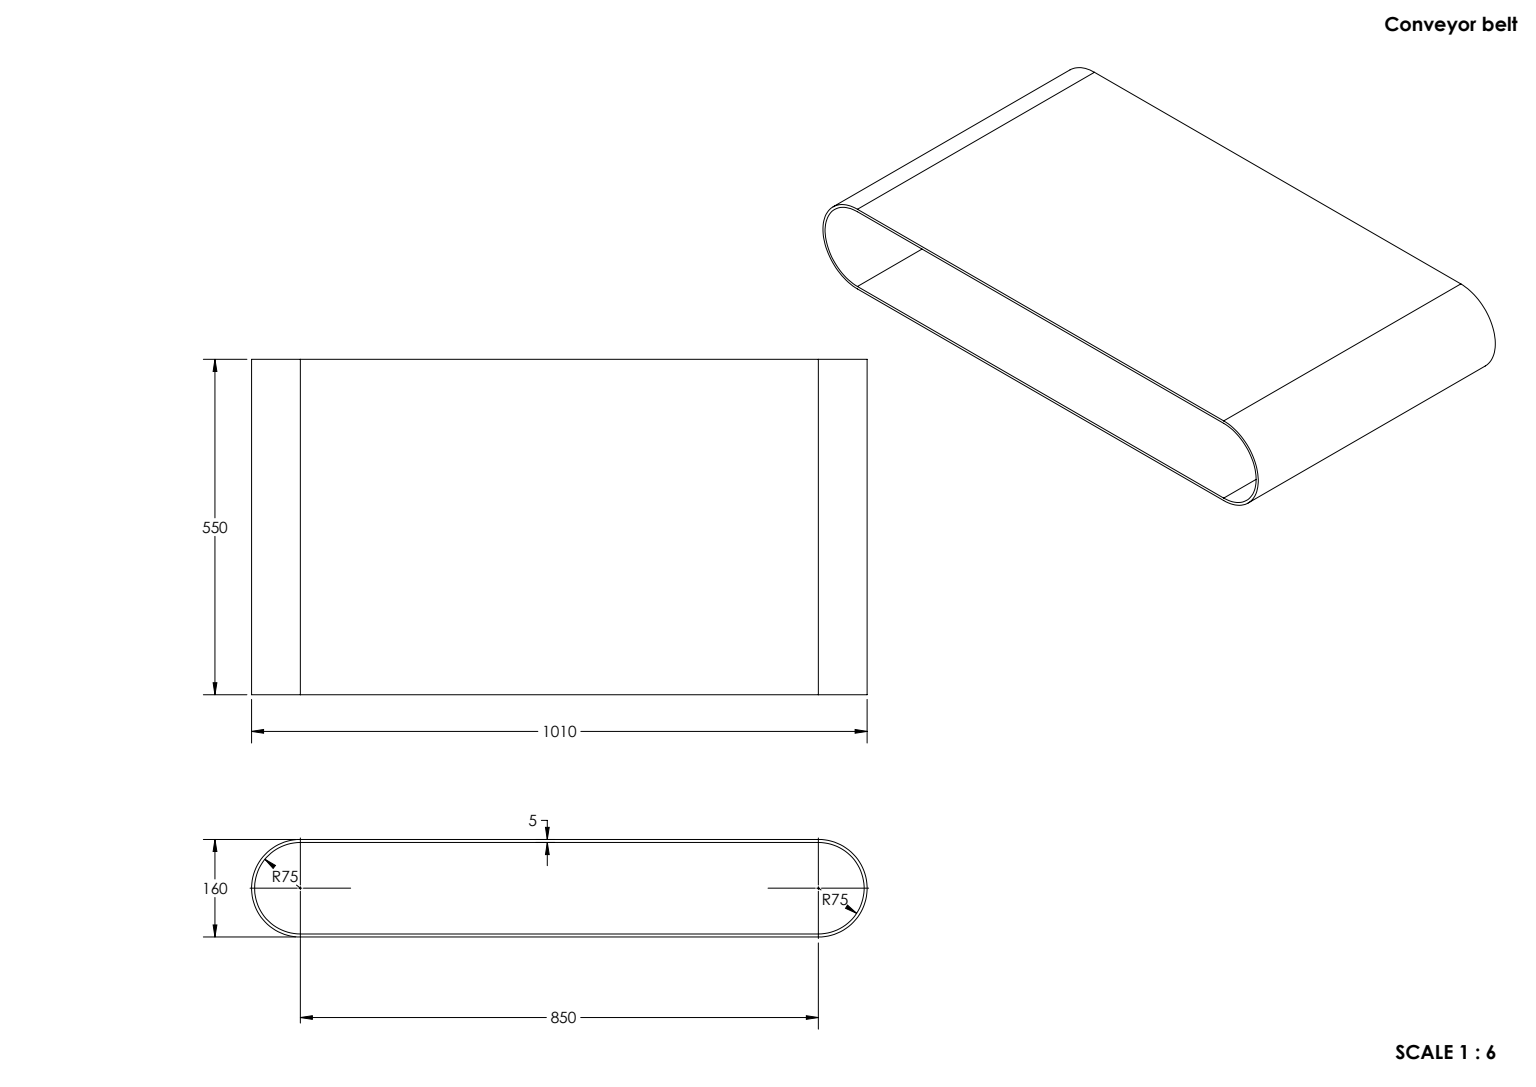
ISO-10303-21;
HEADER;
FILE_DESCRIPTION (('STEP AP214'),
    '1' );
FILE_NAME ('Conveyor belt.step',
    '2026-10-24T15:53:57',
    ( '' ),
    ( '' ),
    'SwSTEP 2.0',
    'SolidWorks 2025',
    '' );
FILE_SCHEMA (( 'AUTOMOTIVE_DESIGN' ));
ENDSEC;

DATA;
#9=LINE ( 'NONE', #1201, #6141 ) ;
#21=VERTEX_POINT ( 'NONE', #2818 ) ;
#37=PRODUCT_CONTEXT ( 'NONE', #2802, 'mechanical' ) ;
#53=CARTESIAN_POINT ( 'NONE',  ( 275.0000000000000000, -425.0000000000000000, 80.00000000000000000 ) ) ;
#85=ORIENTED_EDGE ( 'NONE', *, *, #6307, .F. ) ;
#150=( NAMED_UNIT ( * ) PLANE_ANGLE_UNIT ( ) SI_UNIT ( $, .RADIAN. ) );
#157=CYLINDRICAL_SURFACE ( 'NONE', #5418, 80.00000000000000000 ) ;
#189=AXIS2_PLACEMENT_3D ( 'NONE', #4605, #682, #3336 ) ;
#195=( NAMED_UNIT ( * ) SI_UNIT ( $, .STERADIAN. ) SOLID_ANGLE_UNIT ( ) );
#211=CARTESIAN_POINT ( 'NONE',  ( -275.0000000000000000, -425.0000000000000000, 75.00000000000000000 ) ) ;
#230=ADVANCED_BREP_SHAPE_REPRESENTATION ( '', ( #2980, #7563 ), #1574 ) ;
#257=ORIENTED_EDGE ( 'NONE', *, *, #5557, .F. ) ;
#285=( GEOMETRIC_REPRESENTATION_CONTEXT ( 3 ) GLOBAL_UNCERTAINTY_ASSIGNED_CONTEXT ( ( #4742 ) ) GLOBAL_UNIT_ASSIGNED_CONTEXT ( ( #5304, #150, #6149 ) ) REPRESENTATION_CONTEXT ( 'NONE', 'WORKASPACE' ) );
#287=AXIS2_PLACEMENT_3D ( 'NONE', #7730, #8435, #429 ) ;
#329=ORIENTED_EDGE ( 'NONE', *, *, #2161, .T. ) ;
#356=VECTOR ( 'NONE', #2554, 1000.000000000000000 ) ;
#429=DIRECTION ( 'NONE',  ( 0.000000000000000000, 0.000000000000000000, -1.000000000000000000 ) ) ;
#443=ORIENTED_EDGE ( 'NONE', *, *, #4512, .F. ) ;
#457=CIRCLE ( 'NONE', #6440, 80.00000000000001421 ) ;
#520=DIRECTION ( 'NONE',  ( 0.000000000000000000, 0.000000000000000000, -1.000000000000000000 ) ) ;
#571=EDGE_CURVE ( 'NONE', #3965, #8336, #5577, .T. ) ;
#579=VERTEX_POINT ( 'NONE', #822 ) ;
#614=CARTESIAN_POINT ( 'NONE',  ( 275.0000000000000000, 425.0000000000000000, 1.561424668912875158E-13 ) ) ;
#620=SHAPE_DEFINITION_REPRESENTATION ( #629, #5209 ) ;
#629=PRODUCT_DEFINITION_SHAPE ( 'NONE', 'NONE',  #2753 ) ;
#644=CARTESIAN_POINT ( 'NONE',  ( -275.0000000000000000, 425.0000000000000000, 75.00000000000015632 ) ) ;
#682=DIRECTION ( 'NONE',  ( -1.000000000000000000, -0.000000000000000000, -0.000000000000000000 ) ) ;
#684=ADVANCED_FACE ( 'NONE', ( #8308 ), #1670, .T. ) ;
#700=DIRECTION ( 'NONE',  ( -1.000000000000000000, -0.000000000000000000, -0.000000000000000000 ) ) ;
#793=CIRCLE ( 'NONE', #2448, 80.00000000000001421 ) ;
#804=ORIENTED_EDGE ( 'NONE', *, *, #5681, .F. ) ;
#822=CARTESIAN_POINT ( 'NONE',  ( 275.0000000000000000, 425.0000000000000000, -74.99999999999984368 ) ) ;
#828=VERTEX_POINT ( 'NONE', #1919 ) ;
#852=DIRECTION ( 'NONE',  ( 1.000000000000000000, 0.000000000000000000, 0.000000000000000000 ) ) ;
#877=DIRECTION ( 'NONE',  ( -1.000000000000000000, -0.000000000000000000, -0.000000000000000000 ) ) ;
#897=AXIS2_PLACEMENT_3D ( 'NONE', #2889, #852, #2808 ) ;
#937=FACE_OUTER_BOUND ( 'NONE', #8273, .T. ) ;
#966=VECTOR ( 'NONE', #3191, 1000.000000000000000 ) ;
#975=CARTESIAN_POINT ( 'NONE',  ( 275.0000000000000000, -425.0000000000000000, 80.00000000000000000 ) ) ;
#985=EDGE_CURVE ( 'NONE', #2467, #3965, #3106, .T. ) ;
#1037=ORIENTED_EDGE ( 'NONE', *, *, #5557, .T. ) ;
#1062=EDGE_CURVE ( 'NONE', #828, #3789, #4177, .T. ) ;
#1077=ADVANCED_FACE ( 'NONE', ( #2263 ), #4920, .T. ) ;
#1090=PLANE ( 'NONE',  #1105 ) ;
#1105=AXIS2_PLACEMENT_3D ( 'NONE', #1685, #4478, #520 ) ;
#1121=DIRECTION ( 'NONE',  ( 0.000000000000000000, -1.000000000000000000, -1.795949010423047620E-16 ) ) ;
#1122=EDGE_LOOP ( 'NONE', ( #2153, #1445, #329, #3321 ) ) ;
#1124=EDGE_CURVE ( 'NONE', #8386, #828, #1181, .T. ) ;
#1168=FACE_OUTER_BOUND ( 'NONE', #1171, .T. ) ;
#1171=EDGE_LOOP ( 'NONE', ( #804, #4109, #3770, #257 ) ) ;
#1181=CIRCLE ( 'NONE', #6081, 80.00000000000001421 ) ;
#1193=VECTOR ( 'NONE', #3510, 1000.000000000000000 ) ;
#1201=CARTESIAN_POINT ( 'NONE',  ( 275.0000000000000000, 425.0000000000000000, 80.00000000000015632 ) ) ;
#1283=PLANE ( 'NONE',  #3713 ) ;
#1286=CARTESIAN_POINT ( 'NONE',  ( -275.0000000000000000, -425.0000000000000000, -75.00000000000000000 ) ) ;
#1328=EDGE_CURVE ( 'NONE', #828, #6748, #1386, .T. ) ;
#1339=UNCERTAINTY_MEASURE_WITH_UNIT (LENGTH_MEASURE( 1.000000000000000082E-05 ), #2325, 'distance_accuracy_value', 'NONE');
#1369=ORIENTED_EDGE ( 'NONE', *, *, #4136, .F. ) ;
#1386=LINE ( 'NONE', #4044, #8427 ) ;
#1426=LINE ( 'NONE', #2771, #1193 ) ;
#1436=ORIENTED_EDGE ( 'NONE', *, *, #5113, .F. ) ;
#1445=ORIENTED_EDGE ( 'NONE', *, *, #8307, .F. ) ;
#1526=EDGE_CURVE ( 'NONE', #6748, #2467, #4507, .T. ) ;
#1574=( GEOMETRIC_REPRESENTATION_CONTEXT ( 3 ) GLOBAL_UNCERTAINTY_ASSIGNED_CONTEXT ( ( #1339 ) ) GLOBAL_UNIT_ASSIGNED_CONTEXT ( ( #2325, #6916, #195 ) ) REPRESENTATION_CONTEXT ( 'NONE', 'WORKASPACE' ) );
#1576=AXIS2_PLACEMENT_3D ( 'NONE', #7579, #7742, #2468 ) ;
#1581=ORIENTED_EDGE ( 'NONE', *, *, #5507, .T. ) ;
#1595=DIRECTION ( 'NONE',  ( 0.000000000000000000, -1.000000000000000000, -1.795949010423047620E-16 ) ) ;
#1600=ORIENTED_EDGE ( 'NONE', *, *, #1062, .F. ) ;
#1609=VECTOR ( 'NONE', #4423, 1000.000000000000000 ) ;
#1670=CYLINDRICAL_SURFACE ( 'NONE', #5189, 80.00000000000000000 ) ;
#1676=CARTESIAN_POINT ( 'NONE',  ( 275.0000000000000000, 425.0000000000000000, 75.00000000000015632 ) ) ;
#1685=CARTESIAN_POINT ( 'NONE',  ( -275.0000000000000000, -425.0000000000000000, 0.000000000000000000 ) ) ;
#1755=ADVANCED_FACE ( 'NONE', ( #2731 ), #1283, .F. ) ;
#1858=VECTOR ( 'NONE', #877, 1000.000000000000000 ) ;
#1868=EDGE_LOOP ( 'NONE', ( #443, #5994, #2835, #8154 ) ) ;
#1919=CARTESIAN_POINT ( 'NONE',  ( 275.0000000000000000, -425.0000000000000000, -80.00000000000000000 ) ) ;
#1994=CARTESIAN_POINT ( 'NONE',  ( -275.0000000000000000, -425.0000000000000000, 0.000000000000000000 ) ) ;
#2043=ORIENTED_EDGE ( 'NONE', *, *, #5848, .T. ) ;
#2051=EDGE_CURVE ( 'NONE', #2597, #579, #5794, .T. ) ;
#2153=ORIENTED_EDGE ( 'NONE', *, *, #2377, .F. ) ;
#2161=EDGE_CURVE ( 'NONE', #4536, #8239, #6044, .T. ) ;
#2203=ORIENTED_EDGE ( 'NONE', *, *, #3116, .T. ) ;
#2206=SHAPE_REPRESENTATION_RELATIONSHIP ( 'NONE' , 'NONE' ,  #5209, #230 ) ;
#2226=EDGE_CURVE ( 'NONE', #8239, #3300, #5651, .T. ) ;
#2227=CARTESIAN_POINT ( 'NONE',  ( 275.0000000000000000, 425.0000000000000000, 75.00000000000015632 ) ) ;
#2229=STYLED_ITEM('',(#8670),#2980);
#2257=EDGE_LOOP ( 'NONE', ( #2795, #7341, #6442, #2605 ) ) ;
#2263=FACE_OUTER_BOUND ( 'NONE', #1122, .T. ) ;
#2296=DIRECTION ( 'NONE',  ( 0.000000000000000000, 0.000000000000000000, 1.000000000000000000 ) ) ;
#2325=( LENGTH_UNIT ( ) NAMED_UNIT ( * ) SI_UNIT ( .MILLI., .METRE. ) );
#2358=FACE_OUTER_BOUND ( 'NONE', #2257, .T. ) ;
#2359=VECTOR ( 'NONE', #8298, 1000.000000000000000 ) ;
#2377=EDGE_CURVE ( 'NONE', #5689, #3300, #4968, .T. ) ;
#2388=ORIENTED_EDGE ( 'NONE', *, *, #985, .T. ) ;
#2448=AXIS2_PLACEMENT_3D ( 'NONE', #1994, #4561, #2518 ) ;
#2467=VERTEX_POINT ( 'NONE', #8202 ) ;
#2468=DIRECTION ( 'NONE',  ( 0.000000000000000000, 1.000000000000000000, 1.795949010423047374E-16 ) ) ;
#2474=EDGE_CURVE ( 'NONE', #6426, #8386, #6945, .T. ) ;
#2478=DIRECTION ( 'NONE',  ( 0.000000000000000000, 0.000000000000000000, -1.000000000000000000 ) ) ;
#2518=DIRECTION ( 'NONE',  ( 0.000000000000000000, 1.000000000000000000, 0.000000000000000000 ) ) ;
#2519=ADVANCED_FACE ( 'NONE', ( #2804 ), #3500, .T. ) ;
#2554=DIRECTION ( 'NONE',  ( 0.000000000000000000, 1.000000000000000000, 1.795949010423047374E-16 ) ) ;
#2589=ORIENTED_EDGE ( 'NONE', *, *, #2474, .F. ) ;
#2597=VERTEX_POINT ( 'NONE', #3720 ) ;
#2605=ORIENTED_EDGE ( 'NONE', *, *, #4352, .T. ) ;
#2612=DIRECTION ( 'NONE',  ( 1.000000000000000000, 0.000000000000000000, 0.000000000000000000 ) ) ;
#2625=ORIENTED_EDGE ( 'NONE', *, *, #4808, .F. ) ;
#2660=LINE ( 'NONE', #7836, #7682 ) ;
#2661=ORIENTED_EDGE ( 'NONE', *, *, #3116, .F. ) ;
#2690=CYLINDRICAL_SURFACE ( 'NONE', #189, 75.00000000000000000 ) ;
#2708=LINE ( 'NONE', #7274, #6315 ) ;
#2719=CARTESIAN_POINT ( 'NONE',  ( 275.0000000000000000, -425.0000000000000000, 75.00000000000000000 ) ) ;
#2720=ORIENTED_EDGE ( 'NONE', *, *, #4512, .T. ) ;
#2731=FACE_OUTER_BOUND ( 'NONE', #8566, .T. ) ;
#2753=PRODUCT_DEFINITION ( 'UNKNOWN', '', #8136, #5248 ) ;
#2771=CARTESIAN_POINT ( 'NONE',  ( -275.0000000000000000, -425.0000000000000000, -80.00000000000000000 ) ) ;
#2775=ORIENTED_EDGE ( 'NONE', *, *, #5681, .T. ) ;
#2795=ORIENTED_EDGE ( 'NONE', *, *, #5848, .F. ) ;
#2802=APPLICATION_CONTEXT ( 'automotive_design' ) ;
#2804=FACE_OUTER_BOUND ( 'NONE', #6816, .T. ) ;
#2807=ORIENTED_EDGE ( 'NONE', *, *, #2161, .F. ) ;
#2808=DIRECTION ( 'NONE',  ( 0.000000000000000000, 0.000000000000000000, -1.000000000000000000 ) ) ;
#2818=CARTESIAN_POINT ( 'NONE',  ( -275.0000000000000000, 425.0000000000000000, -74.99999999999984368 ) ) ;
#2835=ORIENTED_EDGE ( 'NONE', *, *, #4808, .T. ) ;
#2853=DIRECTION ( 'NONE',  ( 0.000000000000000000, 1.000000000000000000, 0.000000000000000000 ) ) ;
#2889=CARTESIAN_POINT ( 'NONE',  ( 275.0000000000000000, -425.0000000000000000, 0.000000000000000000 ) ) ;
#2897=ORIENTED_EDGE ( 'NONE', *, *, #571, .T. ) ;
#2949=LINE ( 'NONE', #1676, #4319 ) ;
#2978=VERTEX_POINT ( 'NONE', #3338 ) ;
#2980=MANIFOLD_SOLID_BREP ( 'Extrude-Thin1', #6001 ) ;
#2982=CARTESIAN_POINT ( 'NONE',  ( 275.0000000000000000, -425.0000000000000000, 0.000000000000000000 ) ) ;
#2989=EDGE_LOOP ( 'NONE', ( #8204, #85, #2807, #2625 ) ) ;
#3100=CYLINDRICAL_SURFACE ( 'NONE', #4489, 75.00000000000000000 ) ;
#3106=CIRCLE ( 'NONE', #7421, 80.00000000000001421 ) ;
#3116=EDGE_CURVE ( 'NONE', #8386, #8336, #2660, .T. ) ;
#3175=ORIENTED_EDGE ( 'NONE', *, *, #2051, .T. ) ;
#3191=DIRECTION ( 'NONE',  ( -0.000000000000000000, -1.000000000000000000, -1.795949010423047374E-16 ) ) ;
#3234=VECTOR ( 'NONE', #1595, 1000.000000000000000 ) ;
#3239=APPLICATION_CONTEXT ( 'automotive_design' ) ;
#3293=CIRCLE ( 'NONE', #8170, 75.00000000000000000 ) ;
#3299=CARTESIAN_POINT ( 'NONE',  ( 275.0000000000000000, -425.0000000000000000, 75.00000000000000000 ) ) ;
#3300=VERTEX_POINT ( 'NONE', #211 ) ;
#3321=ORIENTED_EDGE ( 'NONE', *, *, #2226, .T. ) ;
#3335=LINE ( 'NONE', #1286, #356 ) ;
#3336=DIRECTION ( 'NONE',  ( 0.000000000000000000, 0.000000000000000000, 1.000000000000000000 ) ) ;
#3338=CARTESIAN_POINT ( 'NONE',  ( -275.0000000000000000, -425.0000000000000000, -75.00000000000000000 ) ) ;
#3367=ORIENTED_EDGE ( 'NONE', *, *, #5113, .T. ) ;
#3411=DIRECTION ( 'NONE',  ( 1.000000000000000000, 0.000000000000000000, 0.000000000000000000 ) ) ;
#3419=PLANE ( 'NONE',  #897 ) ;
#3477=CARTESIAN_POINT ( 'NONE',  ( 275.0000000000000000, 425.0000000000000000, 1.561424668912875158E-13 ) ) ;
#3491=ORIENTED_EDGE ( 'NONE', *, *, #4136, .T. ) ;
#3500=PLANE ( 'NONE',  #6268 ) ;
#3510=DIRECTION ( 'NONE',  ( 0.000000000000000000, 1.000000000000000000, 1.795949010423047620E-16 ) ) ;
#3512=DIRECTION ( 'NONE',  ( 1.000000000000000000, 0.000000000000000000, 0.000000000000000000 ) ) ;
#3514=ORIENTED_EDGE ( 'NONE', *, *, #4352, .F. ) ;
#3569=DIRECTION ( 'NONE',  ( -1.000000000000000000, -0.000000000000000000, -0.000000000000000000 ) ) ;
#3707=DIRECTION ( 'NONE',  ( 1.000000000000000000, 0.000000000000000000, 0.000000000000000000 ) ) ;
#3713=AXIS2_PLACEMENT_3D ( 'NONE', #53, #7557, #5430 ) ;
#3720=CARTESIAN_POINT ( 'NONE',  ( 275.0000000000000000, -425.0000000000000000, -75.00000000000000000 ) ) ;
#3732=CARTESIAN_POINT ( 'NONE',  ( 275.0000000000000000, -425.0000000000000000, 0.000000000000000000 ) ) ;
#3739=LINE ( 'NONE', #6973, #6896 ) ;
#3770=ORIENTED_EDGE ( 'NONE', *, *, #985, .F. ) ;
#3789=VERTEX_POINT ( 'NONE', #4785 ) ;
#3847=CARTESIAN_POINT ( 'NONE',  ( -275.0000000000000000, 425.0000000000000000, 80.00000000000015632 ) ) ;
#3863=CARTESIAN_POINT ( 'NONE',  ( 275.0000000000000000, 425.0000000000000000, -79.99999999999984368 ) ) ;
#3900=FACE_OUTER_BOUND ( 'NONE', #6229, .T. ) ;
#3906=ORIENTED_EDGE ( 'NONE', *, *, #5444, .T. ) ;
#3926=DIRECTION ( 'NONE',  ( -0.000000000000000000, -1.000000000000000000, -1.795949010423047374E-16 ) ) ;
#3930=CIRCLE ( 'NONE', #6183, 75.00000000000000000 ) ;
#3965=VERTEX_POINT ( 'NONE', #3847 ) ;
#4042=MECHANICAL_DESIGN_GEOMETRIC_PRESENTATION_REPRESENTATION('',(#2229),#285);
#4044=CARTESIAN_POINT ( 'NONE',  ( 275.0000000000000000, -425.0000000000000000, -80.00000000000000000 ) ) ;
#4049=ORIENTED_EDGE ( 'NONE', *, *, #1526, .F. ) ;
#4051=EDGE_LOOP ( 'NONE', ( #2043, #1581, #2720, #5798 ) ) ;
#4106=ADVANCED_FACE ( 'NONE', ( #937, #5559 ), #3419, .T. ) ;
#4109=ORIENTED_EDGE ( 'NONE', *, *, #571, .F. ) ;
#4136=EDGE_CURVE ( 'NONE', #6748, #6426, #457, .T. ) ;
#4170=DIRECTION ( 'NONE',  ( -1.000000000000000000, -0.000000000000000000, -0.000000000000000000 ) ) ;
#4177=LINE ( 'NONE', #6848, #1858 ) ;
#4198=ADVANCED_FACE ( 'NONE', ( #2358 ), #3100, .F. ) ;
#4203=CARTESIAN_POINT ( 'NONE',  ( 0.000000000000000000, 0.000000000000000000, 0.000000000000000000 ) ) ;
#4307=ORIENTED_EDGE ( 'NONE', *, *, #1526, .T. ) ;
#4319=VECTOR ( 'NONE', #4170, 1000.000000000000000 ) ;
#4352=EDGE_CURVE ( 'NONE', #2597, #2978, #2708, .T. ) ;
#4407=DIRECTION ( 'NONE',  ( -1.000000000000000000, -0.000000000000000000, -0.000000000000000000 ) ) ;
#4423=DIRECTION ( 'NONE',  ( -1.000000000000000000, -0.000000000000000000, -0.000000000000000000 ) ) ;
#4428=CARTESIAN_POINT ( 'NONE',  ( 275.0000000000000000, -425.0000000000000000, -80.00000000000000000 ) ) ;
#4445=ORIENTED_EDGE ( 'NONE', *, *, #1328, .F. ) ;
#4478=DIRECTION ( 'NONE',  ( 1.000000000000000000, 0.000000000000000000, 0.000000000000000000 ) ) ;
#4489=AXIS2_PLACEMENT_3D ( 'NONE', #2982, #6385, #5018 ) ;
#4495=CARTESIAN_POINT ( 'NONE',  ( 275.0000000000000000, -425.0000000000000000, -75.00000000000000000 ) ) ;
#4507=LINE ( 'NONE', #7010, #1609 ) ;
#4512=EDGE_CURVE ( 'NONE', #21, #5689, #5049, .T. ) ;
#4534=CARTESIAN_POINT ( 'NONE',  ( 275.0000000000000000, -425.0000000000000000, 0.000000000000000000 ) ) ;
#4536=VERTEX_POINT ( 'NONE', #2227 ) ;
#4561=DIRECTION ( 'NONE',  ( 1.000000000000000000, 0.000000000000000000, 0.000000000000000000 ) ) ;
#4605=CARTESIAN_POINT ( 'NONE',  ( 275.0000000000000000, 425.0000000000000000, 1.561424668912875158E-13 ) ) ;
#4662=ORIENTED_EDGE ( 'NONE', *, *, #2474, .T. ) ;
#4742=UNCERTAINTY_MEASURE_WITH_UNIT (LENGTH_MEASURE( 1.000000000000000082E-05 ), #5304, 'distance_accuracy_value', 'NONE');
#4785=CARTESIAN_POINT ( 'NONE',  ( -275.0000000000000000, -425.0000000000000000, -80.00000000000000000 ) ) ;
#4787=AXIS2_PLACEMENT_3D ( 'NONE', #6634, #3411, #6724 ) ;
#4808=EDGE_CURVE ( 'NONE', #579, #4536, #3293, .T. ) ;
#4828=CARTESIAN_POINT ( 'NONE',  ( 275.0000000000000000, -425.0000000000000000, 80.00000000000000000 ) ) ;
#4889=DIRECTION ( 'NONE',  ( 0.000000000000000000, -1.000000000000000000, -1.795949010423047620E-16 ) ) ;
#4920=PLANE ( 'NONE',  #1576 ) ;
#4968=LINE ( 'NONE', #7629, #966 ) ;
#4998=CARTESIAN_POINT ( 'NONE',  ( -275.0000000000000000, 425.0000000000000000, 1.561424668912875158E-13 ) ) ;
#5003=ORIENTED_EDGE ( 'NONE', *, *, #1062, .T. ) ;
#5007=VECTOR ( 'NONE', #4407, 1000.000000000000000 ) ;
#5018=DIRECTION ( 'NONE',  ( 0.000000000000000000, 0.000000000000000000, 1.000000000000000000 ) ) ;
#5049=CIRCLE ( 'NONE', #4787, 75.00000000000000000 ) ;
#5070=ORIENTED_EDGE ( 'NONE', *, *, #5507, .F. ) ;
#5113=EDGE_CURVE ( 'NONE', #6426, #3965, #9, .T. ) ;
#5189=AXIS2_PLACEMENT_3D ( 'NONE', #3732, #5718, #6396 ) ;
#5209=SHAPE_REPRESENTATION ( 'Conveyor belt', ( #7563 ), #1574 ) ;
#5248=PRODUCT_DEFINITION_CONTEXT ( 'detailed design', #3239, 'design' ) ;
#5272=EDGE_LOOP ( 'NONE', ( #2775, #1600, #7986, #2203 ) ) ;
#5294=ADVANCED_FACE ( 'NONE', ( #1168, #7791 ), #1090, .F. ) ;
#5304=( LENGTH_UNIT ( ) NAMED_UNIT ( * ) SI_UNIT ( .MILLI., .METRE. ) );
#5418=AXIS2_PLACEMENT_3D ( 'NONE', #3477, #3569, #2296 ) ;
#5426=DIRECTION ( 'NONE',  ( 1.000000000000000000, 0.000000000000000000, 0.000000000000000000 ) ) ;
#5430=DIRECTION ( 'NONE',  ( 0.000000000000000000, 1.000000000000000000, 1.795949010423047620E-16 ) ) ;
#5432=EDGE_LOOP ( 'NONE', ( #2388, #1436, #1369, #4307 ) ) ;
#5444=EDGE_CURVE ( 'NONE', #579, #21, #3739, .T. ) ;
#5507=EDGE_CURVE ( 'NONE', #2978, #21, #3335, .T. ) ;
#5557=EDGE_CURVE ( 'NONE', #3789, #2467, #1426, .T. ) ;
#5559=FACE_BOUND ( 'NONE', #2989, .T. ) ;
#5577=LINE ( 'NONE', #8097, #3234 ) ;
#5651=LINE ( 'NONE', #7673, #5007 ) ;
#5681=EDGE_CURVE ( 'NONE', #8336, #3789, #793, .T. ) ;
#5689=VERTEX_POINT ( 'NONE', #644 ) ;
#5718=DIRECTION ( 'NONE',  ( -1.000000000000000000, -0.000000000000000000, -0.000000000000000000 ) ) ;
#5742=ORIENTED_EDGE ( 'NONE', *, *, #1124, .T. ) ;
#5766=ORIENTED_EDGE ( 'NONE', *, *, #1328, .T. ) ;
#5794=LINE ( 'NONE', #4495, #2359 ) ;
#5798=ORIENTED_EDGE ( 'NONE', *, *, #2377, .T. ) ;
#5848=EDGE_CURVE ( 'NONE', #3300, #2978, #5876, .T. ) ;
#5876=CIRCLE ( 'NONE', #287, 75.00000000000000000 ) ;
#5939=PRODUCT ( 'Conveyor belt', 'Conveyor belt', '', ( #37 ) ) ;
#5994=ORIENTED_EDGE ( 'NONE', *, *, #5444, .F. ) ;
#6001=CLOSED_SHELL ( 'NONE', ( #4106, #5294, #684, #8494, #6952, #1755, #4198, #2519, #8547, #1077 ) ) ;
#6044=LINE ( 'NONE', #2719, #6517 ) ;
#6081=AXIS2_PLACEMENT_3D ( 'NONE', #6478, #3707, #8521 ) ;
#6137=VECTOR ( 'NONE', #4889, 1000.000000000000000 ) ;
#6141=VECTOR ( 'NONE', #6700, 1000.000000000000000 ) ;
#6149=( NAMED_UNIT ( * ) SI_UNIT ( $, .STERADIAN. ) SOLID_ANGLE_UNIT ( ) );
#6173=DIRECTION ( 'NONE',  ( 0.000000000000000000, -1.795949010423047374E-16, 1.000000000000000000 ) ) ;
#6183=AXIS2_PLACEMENT_3D ( 'NONE', #4534, #6534, #8576 ) ;
#6217=CARTESIAN_POINT ( 'NONE',  ( 275.0000000000000000, -425.0000000000000000, -75.00000000000000000 ) ) ;
#6229=EDGE_LOOP ( 'NONE', ( #1037, #4049, #4445, #5003 ) ) ;
#6268=AXIS2_PLACEMENT_3D ( 'NONE', #6217, #6173, #8162 ) ;
#6307=EDGE_CURVE ( 'NONE', #8239, #2597, #3930, .T. ) ;
#6315=VECTOR ( 'NONE', #700, 1000.000000000000000 ) ;
#6331=DIRECTION ( 'NONE',  ( 1.000000000000000000, 0.000000000000000000, 0.000000000000000000 ) ) ;
#6385=DIRECTION ( 'NONE',  ( -1.000000000000000000, -0.000000000000000000, -0.000000000000000000 ) ) ;
#6396=DIRECTION ( 'NONE',  ( 0.000000000000000000, 0.000000000000000000, 1.000000000000000000 ) ) ;
#6426=VERTEX_POINT ( 'NONE', #7459 ) ;
#6440=AXIS2_PLACEMENT_3D ( 'NONE', #8208, #5426, #2853 ) ;
#6442=ORIENTED_EDGE ( 'NONE', *, *, #6307, .T. ) ;
#6478=CARTESIAN_POINT ( 'NONE',  ( 275.0000000000000000, -425.0000000000000000, 0.000000000000000000 ) ) ;
#6517=VECTOR ( 'NONE', #3926, 1000.000000000000000 ) ;
#6534=DIRECTION ( 'NONE',  ( 1.000000000000000000, 0.000000000000000000, 0.000000000000000000 ) ) ;
#6589=AXIS2_PLACEMENT_3D ( 'NONE', #4428, #7089, #1121 ) ;
#6634=CARTESIAN_POINT ( 'NONE',  ( -275.0000000000000000, 425.0000000000000000, 1.561424668912875158E-13 ) ) ;
#6651=FACE_OUTER_BOUND ( 'NONE', #1868, .T. ) ;
#6700=DIRECTION ( 'NONE',  ( -1.000000000000000000, -0.000000000000000000, -0.000000000000000000 ) ) ;
#6702=DIRECTION ( 'NONE',  ( 0.000000000000000000, 1.000000000000000000, 1.795949010423047620E-16 ) ) ;
#6724=DIRECTION ( 'NONE',  ( 0.000000000000000000, 0.000000000000000000, -1.000000000000000000 ) ) ;
#6748=VERTEX_POINT ( 'NONE', #3863 ) ;
#6816=EDGE_LOOP ( 'NONE', ( #5070, #3514, #3175, #3906 ) ) ;
#6848=CARTESIAN_POINT ( 'NONE',  ( 275.0000000000000000, -425.0000000000000000, -80.00000000000000000 ) ) ;
#6896=VECTOR ( 'NONE', #7129, 1000.000000000000000 ) ;
#6916=( NAMED_UNIT ( * ) PLANE_ANGLE_UNIT ( ) SI_UNIT ( $, .RADIAN. ) );
#6945=LINE ( 'NONE', #975, #6137 ) ;
#6952=ADVANCED_FACE ( 'NONE', ( #7572 ), #157, .T. ) ;
#6973=CARTESIAN_POINT ( 'NONE',  ( 275.0000000000000000, 425.0000000000000000, -74.99999999999984368 ) ) ;
#7010=CARTESIAN_POINT ( 'NONE',  ( 275.0000000000000000, 425.0000000000000000, -79.99999999999984368 ) ) ;
#7089=DIRECTION ( 'NONE',  ( 0.000000000000000000, -1.795949010423047620E-16, 1.000000000000000000 ) ) ;
#7129=DIRECTION ( 'NONE',  ( -1.000000000000000000, -0.000000000000000000, -0.000000000000000000 ) ) ;
#7226=DIRECTION ( 'NONE',  ( -1.000000000000000000, -0.000000000000000000, -0.000000000000000000 ) ) ;
#7274=CARTESIAN_POINT ( 'NONE',  ( 275.0000000000000000, -425.0000000000000000, -75.00000000000000000 ) ) ;
#7341=ORIENTED_EDGE ( 'NONE', *, *, #2226, .F. ) ;
#7421=AXIS2_PLACEMENT_3D ( 'NONE', #4998, #6331, #7664 ) ;
#7459=CARTESIAN_POINT ( 'NONE',  ( 275.0000000000000000, 425.0000000000000000, 80.00000000000015632 ) ) ;
#7478=DIRECTION ( 'NONE',  ( 0.000000000000000000, 0.000000000000000000, 1.000000000000000000 ) ) ;
#7557=DIRECTION ( 'NONE',  ( 0.000000000000000000, 1.795949010423047620E-16, -1.000000000000000000 ) ) ;
#7563=AXIS2_PLACEMENT_3D ( 'NONE', #4203, #7478, #3512 ) ;
#7572=FACE_OUTER_BOUND ( 'NONE', #5432, .T. ) ;
#7579=CARTESIAN_POINT ( 'NONE',  ( 275.0000000000000000, -425.0000000000000000, 75.00000000000000000 ) ) ;
#7629=CARTESIAN_POINT ( 'NONE',  ( -275.0000000000000000, -425.0000000000000000, 75.00000000000000000 ) ) ;
#7664=DIRECTION ( 'NONE',  ( 0.000000000000000000, 1.000000000000000000, 0.000000000000000000 ) ) ;
#7673=CARTESIAN_POINT ( 'NONE',  ( 275.0000000000000000, -425.0000000000000000, 75.00000000000000000 ) ) ;
#7682=VECTOR ( 'NONE', #7226, 1000.000000000000000 ) ;
#7730=CARTESIAN_POINT ( 'NONE',  ( -275.0000000000000000, -425.0000000000000000, 0.000000000000000000 ) ) ;
#7742=DIRECTION ( 'NONE',  ( 0.000000000000000000, 1.795949010423047374E-16, -1.000000000000000000 ) ) ;
#7791=FACE_BOUND ( 'NONE', #4051, .T. ) ;
#7836=CARTESIAN_POINT ( 'NONE',  ( 275.0000000000000000, -425.0000000000000000, 80.00000000000000000 ) ) ;
#7986=ORIENTED_EDGE ( 'NONE', *, *, #1124, .F. ) ;
#8097=CARTESIAN_POINT ( 'NONE',  ( -275.0000000000000000, -425.0000000000000000, 80.00000000000000000 ) ) ;
#8136=PRODUCT_DEFINITION_FORMATION_WITH_SPECIFIED_SOURCE ( 'ANY', '', #5939, .NOT_KNOWN. ) ;
#8154=ORIENTED_EDGE ( 'NONE', *, *, #8307, .T. ) ;
#8162=DIRECTION ( 'NONE',  ( 0.000000000000000000, -1.000000000000000000, -1.795949010423047374E-16 ) ) ;
#8170=AXIS2_PLACEMENT_3D ( 'NONE', #614, #2612, #2478 ) ;
#8179=CARTESIAN_POINT ( 'NONE',  ( -275.0000000000000000, -425.0000000000000000, 80.00000000000000000 ) ) ;
#8202=CARTESIAN_POINT ( 'NONE',  ( -275.0000000000000000, 425.0000000000000000, -79.99999999999984368 ) ) ;
#8204=ORIENTED_EDGE ( 'NONE', *, *, #2051, .F. ) ;
#8208=CARTESIAN_POINT ( 'NONE',  ( 275.0000000000000000, 425.0000000000000000, 1.561424668912875158E-13 ) ) ;
#8239=VERTEX_POINT ( 'NONE', #3299 ) ;
#8273=EDGE_LOOP ( 'NONE', ( #5742, #5766, #3491, #4662 ) ) ;
#8298=DIRECTION ( 'NONE',  ( 0.000000000000000000, 1.000000000000000000, 1.795949010423047374E-16 ) ) ;
#8307=EDGE_CURVE ( 'NONE', #4536, #5689, #2949, .T. ) ;
#8308=FACE_OUTER_BOUND ( 'NONE', #5272, .T. ) ;
#8336=VERTEX_POINT ( 'NONE', #8179 ) ;
#8355=PLANE ( 'NONE',  #6589 ) ;
#8386=VERTEX_POINT ( 'NONE', #4828 ) ;
#8427=VECTOR ( 'NONE', #6702, 1000.000000000000000 ) ;
#8435=DIRECTION ( 'NONE',  ( 1.000000000000000000, 0.000000000000000000, 0.000000000000000000 ) ) ;
#8494=ADVANCED_FACE ( 'NONE', ( #3900 ), #8355, .F. ) ;
#8521=DIRECTION ( 'NONE',  ( 0.000000000000000000, 1.000000000000000000, 0.000000000000000000 ) ) ;
#8547=ADVANCED_FACE ( 'NONE', ( #6651 ), #2690, .F. ) ;
#8566=EDGE_LOOP ( 'NONE', ( #2897, #2661, #2589, #3367 ) ) ;
#8576=DIRECTION ( 'NONE',  ( 0.000000000000000000, 0.000000000000000000, -1.000000000000000000 ) ) ;
#8664=COLOUR_RGB('Black',0.12,0.14,0.17);
#8665=FILL_AREA_STYLE_COLOUR('',#8664);
#8666=FILL_AREA_STYLE('',(#8665));
#8667=SURFACE_STYLE_FILL_AREA(#8666);
#8668=SURFACE_SIDE_STYLE('',(#8667));
#8669=SURFACE_STYLE_USAGE(.BOTH.,#8668);
#8670=PRESENTATION_STYLE_ASSIGNMENT((#8669));
ENDSEC;
END-ISO-10303-21;
